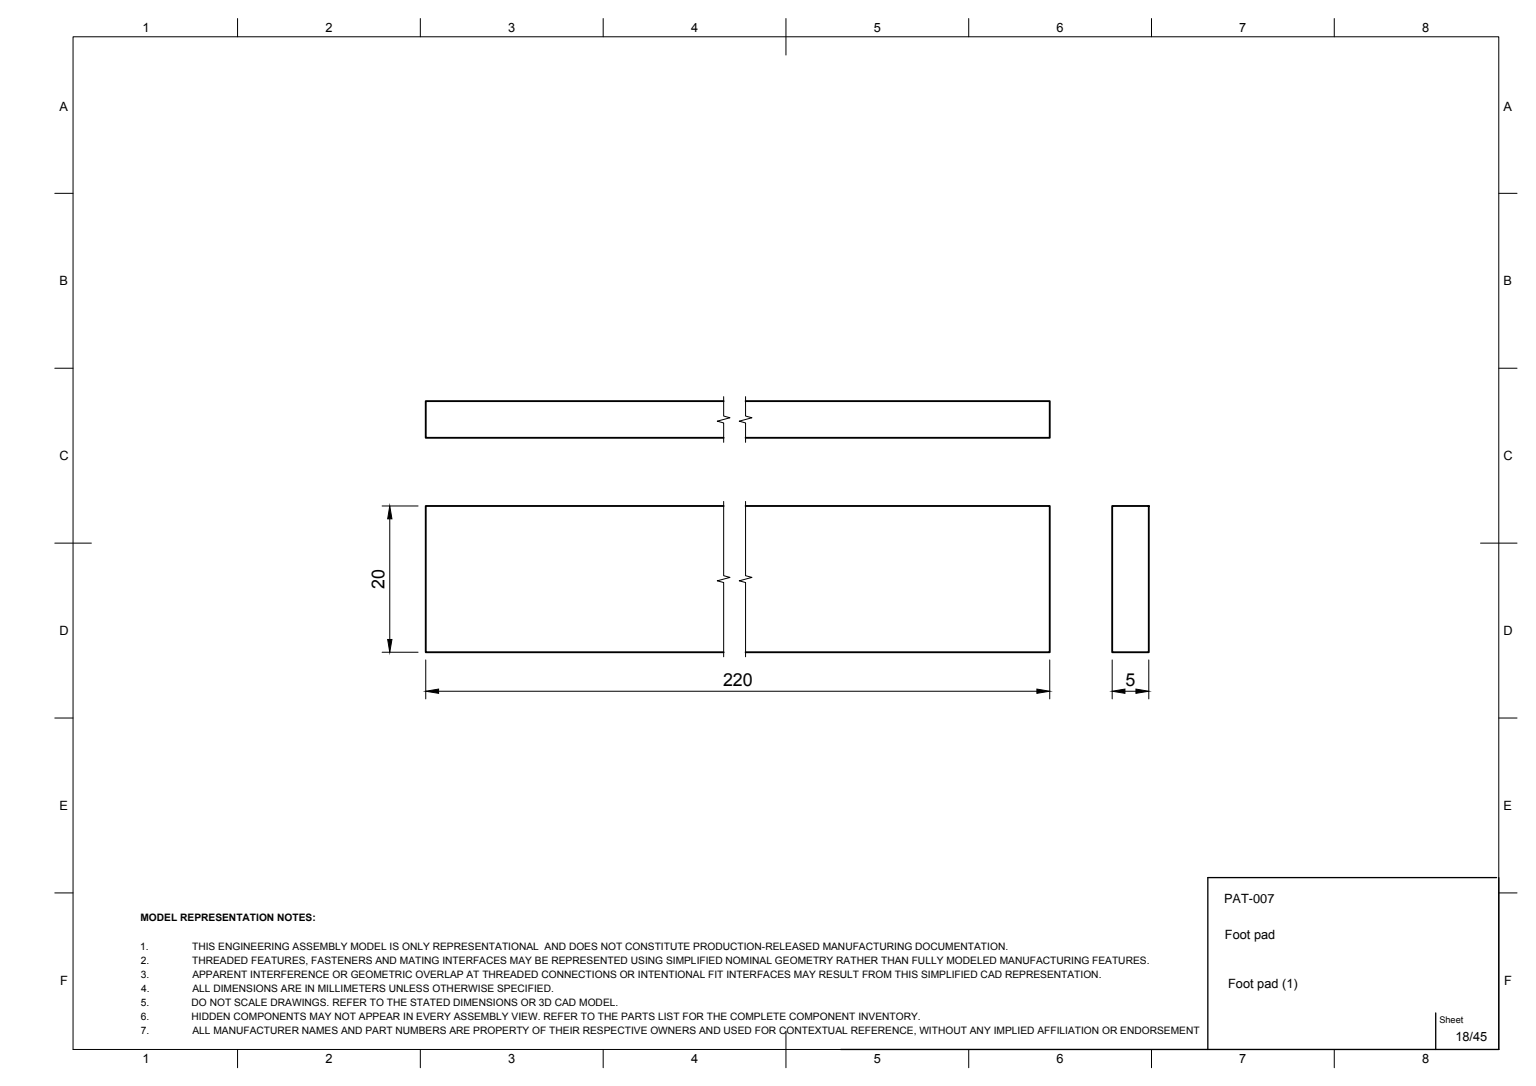
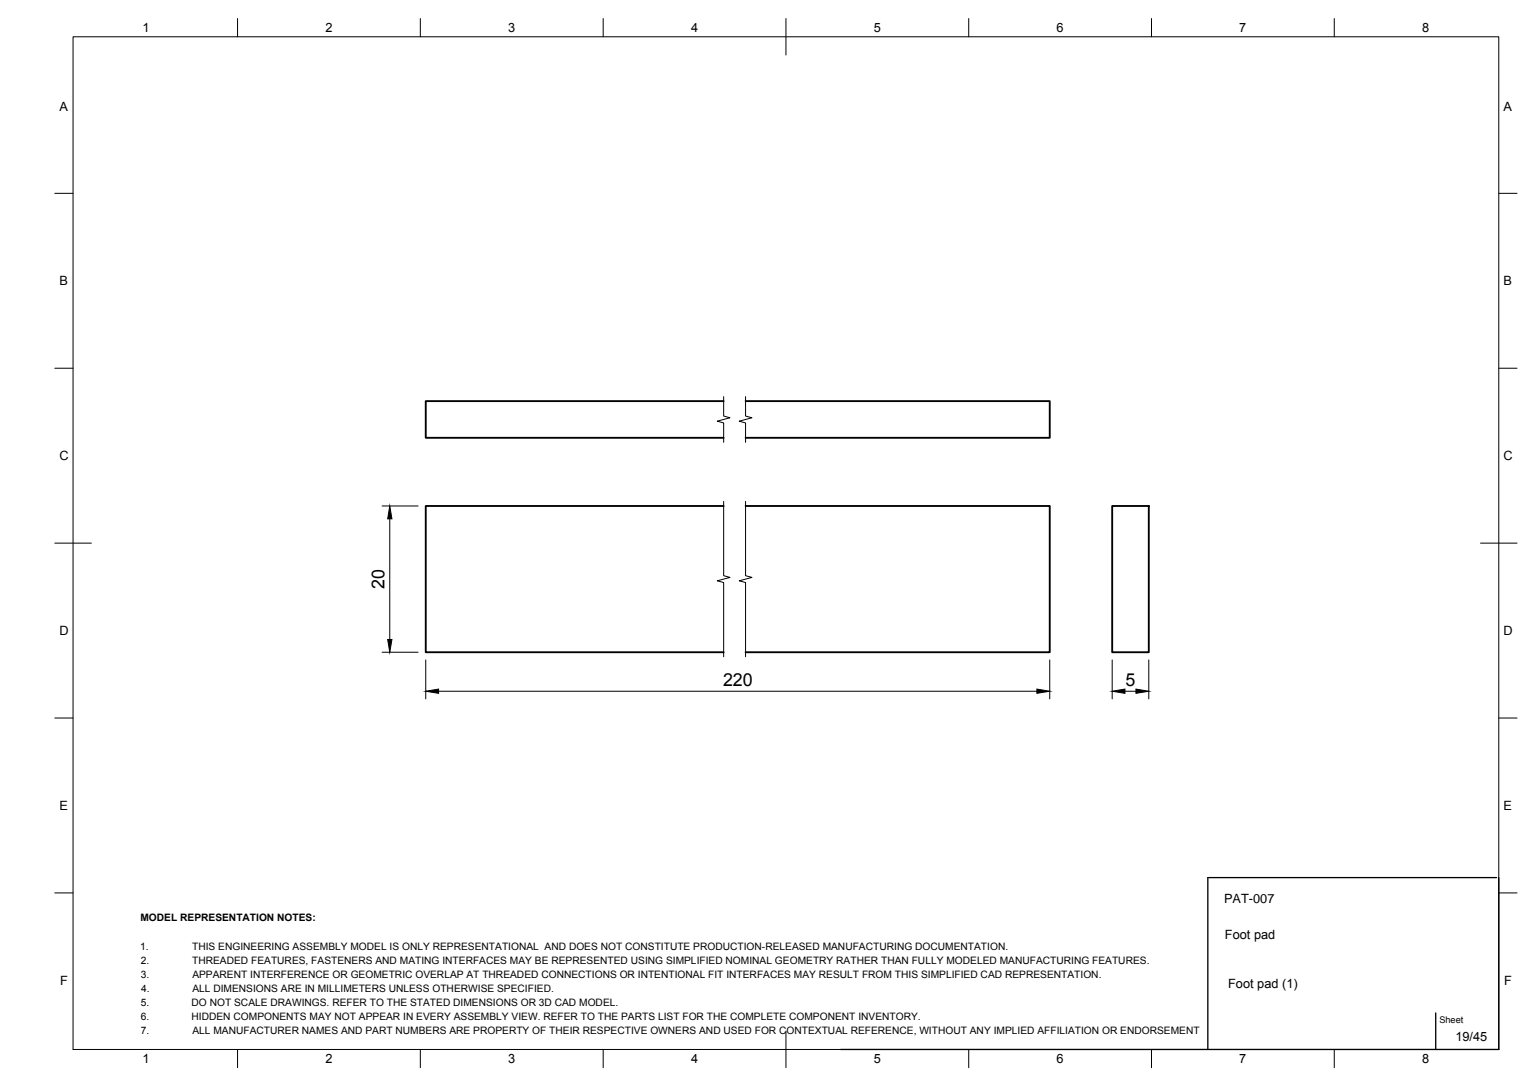
ISO-10303-21;
HEADER;
/* Generated by software containing ST-Developer
 * from STEP Tools, Inc. (www.steptools.com) 
 */

FILE_DESCRIPTION(
/* description */ ('Bearing friction torque test rig'),
/* implementation_level */ '2;1');

FILE_NAME(
/* name */ 'Foot pad.step',
/* time_stamp */ '2026-10-28T03:24:04-07:00',
/* author */ (''),
/* organization */ (''),
/* preprocessor_version */ 'ST-DEVELOPER v20.2',
/* originating_system */ 'Autodesk Translation Framework v15.17.0.0',
/* authorisation */ '');

FILE_SCHEMA (('AUTOMOTIVE_DESIGN { 1 0 10303 214 3 1 1 }'));
ENDSEC;

DATA;
#10=MECHANICAL_DESIGN_GEOMETRIC_PRESENTATION_REPRESENTATION('',(#552),#14822);
#474=SHAPE_REPRESENTATION_RELATIONSHIP('SRR','None',#15013,#513);
#513=ADVANCED_BREP_SHAPE_REPRESENTATION('',(#606),#14793);
#552=STYLED_ITEM('',(#15277),#606);
#606=MANIFOLD_SOLID_BREP('Body1',#7668);
#979=PLANE('',#8585);
#980=PLANE('',#8586);
#981=PLANE('',#8587);
#982=PLANE('',#8588);
#983=PLANE('',#8589);
#984=PLANE('',#8590);
#1308=FACE_OUTER_BOUND('',#1922,.T.);
#1309=FACE_OUTER_BOUND('',#1923,.T.);
#1310=FACE_OUTER_BOUND('',#1924,.T.);
#1311=FACE_OUTER_BOUND('',#1925,.T.);
#1312=FACE_OUTER_BOUND('',#1926,.T.);
#1313=FACE_OUTER_BOUND('',#1927,.T.);
#1922=EDGE_LOOP('',(#6096,#6097,#6098,#6099));
#1923=EDGE_LOOP('',(#6100,#6101,#6102,#6103));
#1924=EDGE_LOOP('',(#6104,#6105,#6106,#6107));
#1925=EDGE_LOOP('',(#6108,#6109,#6110,#6111));
#1926=EDGE_LOOP('',(#6112,#6113,#6114,#6115));
#1927=EDGE_LOOP('',(#6116,#6117,#6118,#6119));
#2475=LINE('',#12676,#2919);
#2476=LINE('',#12678,#2920);
#2477=LINE('',#12680,#2921);
#2478=LINE('',#12681,#2922);
#2479=LINE('',#12684,#2923);
#2480=LINE('',#12686,#2924);
#2481=LINE('',#12687,#2925);
#2482=LINE('',#12690,#2926);
#2483=LINE('',#12692,#2927);
#2484=LINE('',#12693,#2928);
#2485=LINE('',#12695,#2929);
#2486=LINE('',#12696,#2930);
#2919=VECTOR('',#10310,1.);
#2920=VECTOR('',#10311,1.);
#2921=VECTOR('',#10312,1.);
#2922=VECTOR('',#10313,1.);
#2923=VECTOR('',#10316,1.);
#2924=VECTOR('',#10317,1.);
#2925=VECTOR('',#10318,1.);
#2926=VECTOR('',#10321,1.);
#2927=VECTOR('',#10322,1.);
#2928=VECTOR('',#10323,1.);
#2929=VECTOR('',#10326,1.);
#2930=VECTOR('',#10327,1.);
#3869=VERTEX_POINT('',#12674);
#3870=VERTEX_POINT('',#12675);
#3871=VERTEX_POINT('',#12677);
#3872=VERTEX_POINT('',#12679);
#3873=VERTEX_POINT('',#12683);
#3874=VERTEX_POINT('',#12685);
#3875=VERTEX_POINT('',#12689);
#3876=VERTEX_POINT('',#12691);
#4674=EDGE_CURVE('',#3869,#3870,#2475,.T.);
#4675=EDGE_CURVE('',#3870,#3871,#2476,.T.);
#4676=EDGE_CURVE('',#3872,#3871,#2477,.T.);
#4677=EDGE_CURVE('',#3869,#3872,#2478,.T.);
#4678=EDGE_CURVE('',#3873,#3869,#2479,.T.);
#4679=EDGE_CURVE('',#3874,#3872,#2480,.T.);
#4680=EDGE_CURVE('',#3873,#3874,#2481,.T.);
#4681=EDGE_CURVE('',#3875,#3873,#2482,.T.);
#4682=EDGE_CURVE('',#3876,#3874,#2483,.T.);
#4683=EDGE_CURVE('',#3875,#3876,#2484,.T.);
#4684=EDGE_CURVE('',#3870,#3875,#2485,.T.);
#4685=EDGE_CURVE('',#3871,#3876,#2486,.T.);
#6096=ORIENTED_EDGE('',*,*,#4674,.T.);
#6097=ORIENTED_EDGE('',*,*,#4675,.T.);
#6098=ORIENTED_EDGE('',*,*,#4676,.F.);
#6099=ORIENTED_EDGE('',*,*,#4677,.F.);
#6100=ORIENTED_EDGE('',*,*,#4678,.T.);
#6101=ORIENTED_EDGE('',*,*,#4677,.T.);
#6102=ORIENTED_EDGE('',*,*,#4679,.F.);
#6103=ORIENTED_EDGE('',*,*,#4680,.F.);
#6104=ORIENTED_EDGE('',*,*,#4681,.T.);
#6105=ORIENTED_EDGE('',*,*,#4680,.T.);
#6106=ORIENTED_EDGE('',*,*,#4682,.F.);
#6107=ORIENTED_EDGE('',*,*,#4683,.F.);
#6108=ORIENTED_EDGE('',*,*,#4684,.T.);
#6109=ORIENTED_EDGE('',*,*,#4683,.T.);
#6110=ORIENTED_EDGE('',*,*,#4685,.F.);
#6111=ORIENTED_EDGE('',*,*,#4675,.F.);
#6112=ORIENTED_EDGE('',*,*,#4685,.T.);
#6113=ORIENTED_EDGE('',*,*,#4682,.T.);
#6114=ORIENTED_EDGE('',*,*,#4679,.T.);
#6115=ORIENTED_EDGE('',*,*,#4676,.T.);
#6116=ORIENTED_EDGE('',*,*,#4684,.F.);
#6117=ORIENTED_EDGE('',*,*,#4674,.F.);
#6118=ORIENTED_EDGE('',*,*,#4678,.F.);
#6119=ORIENTED_EDGE('',*,*,#4681,.F.);
#7419=ADVANCED_FACE('',(#1308),#979,.T.);
#7420=ADVANCED_FACE('',(#1309),#980,.T.);
#7421=ADVANCED_FACE('',(#1310),#981,.T.);
#7422=ADVANCED_FACE('',(#1311),#982,.T.);
#7423=ADVANCED_FACE('',(#1312),#983,.T.);
#7424=ADVANCED_FACE('',(#1313),#984,.F.);
#7668=CLOSED_SHELL('',(#7419,#7420,#7421,#7422,#7423,#7424));
#8584=AXIS2_PLACEMENT_3D('',#12672,#10306,#10307);
#8585=AXIS2_PLACEMENT_3D('',#12673,#10308,#10309);
#8586=AXIS2_PLACEMENT_3D('',#12682,#10314,#10315);
#8587=AXIS2_PLACEMENT_3D('',#12688,#10319,#10320);
#8588=AXIS2_PLACEMENT_3D('',#12694,#10324,#10325);
#8589=AXIS2_PLACEMENT_3D('',#12697,#10328,#10329);
#8590=AXIS2_PLACEMENT_3D('',#12698,#10330,#10331);
#10306=DIRECTION('axis',(0.,0.,1.));
#10307=DIRECTION('refdir',(1.,0.,0.));
#10308=DIRECTION('center_axis',(0.,1.,0.));
#10309=DIRECTION('ref_axis',(-1.,0.,0.));
#10310=DIRECTION('',(-1.,0.,0.));
#10311=DIRECTION('',(0.,0.,1.));
#10312=DIRECTION('',(-1.,0.,0.));
#10313=DIRECTION('',(0.,0.,1.));
#10314=DIRECTION('center_axis',(1.,0.,0.));
#10315=DIRECTION('ref_axis',(0.,1.,0.));
#10316=DIRECTION('',(0.,1.,0.));
#10317=DIRECTION('',(0.,1.,0.));
#10318=DIRECTION('',(0.,0.,1.));
#10319=DIRECTION('center_axis',(0.,-1.,0.));
#10320=DIRECTION('ref_axis',(1.,0.,0.));
#10321=DIRECTION('',(1.,0.,0.));
#10322=DIRECTION('',(1.,0.,0.));
#10323=DIRECTION('',(0.,0.,1.));
#10324=DIRECTION('center_axis',(-1.,0.,0.));
#10325=DIRECTION('ref_axis',(0.,-1.,0.));
#10326=DIRECTION('',(0.,-1.,0.));
#10327=DIRECTION('',(0.,-1.,0.));
#10328=DIRECTION('center_axis',(0.,0.,1.));
#10329=DIRECTION('ref_axis',(1.,0.,0.));
#10330=DIRECTION('center_axis',(0.,0.,1.));
#10331=DIRECTION('ref_axis',(1.,0.,0.));
#12672=CARTESIAN_POINT('',(0.,0.,0.));
#12673=CARTESIAN_POINT('Origin',(-4.5,11.,-0.5));
#12674=CARTESIAN_POINT('',(-4.5,11.,-0.5));
#12675=CARTESIAN_POINT('',(-6.5,11.,-0.5));
#12676=CARTESIAN_POINT('',(-4.5,11.,-0.5));
#12677=CARTESIAN_POINT('',(-6.5,11.,0.));
#12678=CARTESIAN_POINT('',(-6.5,11.,-0.5));
#12679=CARTESIAN_POINT('',(-4.5,11.,0.));
#12680=CARTESIAN_POINT('',(-4.5,11.,0.));
#12681=CARTESIAN_POINT('',(-4.5,11.,-0.5));
#12682=CARTESIAN_POINT('Origin',(-4.5,-11.,-0.5));
#12683=CARTESIAN_POINT('',(-4.5,-11.,-0.5));
#12684=CARTESIAN_POINT('',(-4.5,-11.,-0.5));
#12685=CARTESIAN_POINT('',(-4.5,-11.,0.));
#12686=CARTESIAN_POINT('',(-4.5,-11.,0.));
#12687=CARTESIAN_POINT('',(-4.5,-11.,-0.5));
#12688=CARTESIAN_POINT('Origin',(-6.5,-11.,-0.5));
#12689=CARTESIAN_POINT('',(-6.5,-11.,-0.5));
#12690=CARTESIAN_POINT('',(-6.5,-11.,-0.5));
#12691=CARTESIAN_POINT('',(-6.5,-11.,0.));
#12692=CARTESIAN_POINT('',(-6.5,-11.,0.));
#12693=CARTESIAN_POINT('',(-6.5,-11.,-0.5));
#12694=CARTESIAN_POINT('Origin',(-6.5,11.,-0.5));
#12695=CARTESIAN_POINT('',(-6.5,11.,-0.5));
#12696=CARTESIAN_POINT('',(-6.5,11.,0.));
#12697=CARTESIAN_POINT('Origin',(-5.5,0.,0.));
#12698=CARTESIAN_POINT('Origin',(-5.5,0.,-0.5));
#14748=UNCERTAINTY_MEASURE_WITH_UNIT(LENGTH_MEASURE(0.001),#14823,
'DISTANCE_ACCURACY_VALUE',
'Maximum model space distance between geometric entities at asserted c
onnectivities');
#14777=UNCERTAINTY_MEASURE_WITH_UNIT(LENGTH_MEASURE(0.001),#14823,
'DISTANCE_ACCURACY_VALUE',
'Maximum model space distance between geometric entities at asserted c
onnectivities');
#14793=(
GEOMETRIC_REPRESENTATION_CONTEXT(3)
GLOBAL_UNCERTAINTY_ASSIGNED_CONTEXT((#14748))
GLOBAL_UNIT_ASSIGNED_CONTEXT((#14823,#14825,#14826))
REPRESENTATION_CONTEXT('','3D')
);
#14822=(
GEOMETRIC_REPRESENTATION_CONTEXT(3)
GLOBAL_UNCERTAINTY_ASSIGNED_CONTEXT((#14777))
GLOBAL_UNIT_ASSIGNED_CONTEXT((#14823,#14825,#14826))
REPRESENTATION_CONTEXT('','3D')
);
#14823=(
LENGTH_UNIT()
NAMED_UNIT(*)
SI_UNIT(.CENTI.,.METRE.)
);
#14825=(
NAMED_UNIT(*)
PLANE_ANGLE_UNIT()
SI_UNIT($,.RADIAN.)
);
#14826=(
NAMED_UNIT(*)
SI_UNIT($,.STERADIAN.)
SOLID_ANGLE_UNIT()
);
#14842=SHAPE_DEFINITION_REPRESENTATION(#14886,#15013);
#14886=PRODUCT_DEFINITION_SHAPE('',$,#15058);
#15013=SHAPE_REPRESENTATION('',(#8584),#14793);
#15042=PRODUCT_DEFINITION_CONTEXT('part definition',#15176,'design');
#15058=PRODUCT_DEFINITION('Foot pad','Foot pad',#15102,#15042);
#15102=PRODUCT_DEFINITION_FORMATION('',$,#15193);
#15176=APPLICATION_CONTEXT(
'Core Data for Automotive Mechanical Design Process');
#15177=PRODUCT_CONTEXT('part definition',#15176,'mechanical');
#15193=PRODUCT('Foot pad','Foot pad','Foot pad',(#15177));
#15271=COLOUR_RGB('Sky Blue',0.24,0.69,0.87);
#15272=FILL_AREA_STYLE_COLOUR('',#15271);
#15273=FILL_AREA_STYLE('',(#15272));
#15274=SURFACE_STYLE_FILL_AREA(#15273);
#15275=SURFACE_SIDE_STYLE('',(#15274));
#15276=SURFACE_STYLE_USAGE(.BOTH.,#15275);
#15277=PRESENTATION_STYLE_ASSIGNMENT((#15276));
ENDSEC;
END-ISO-10303-21;
